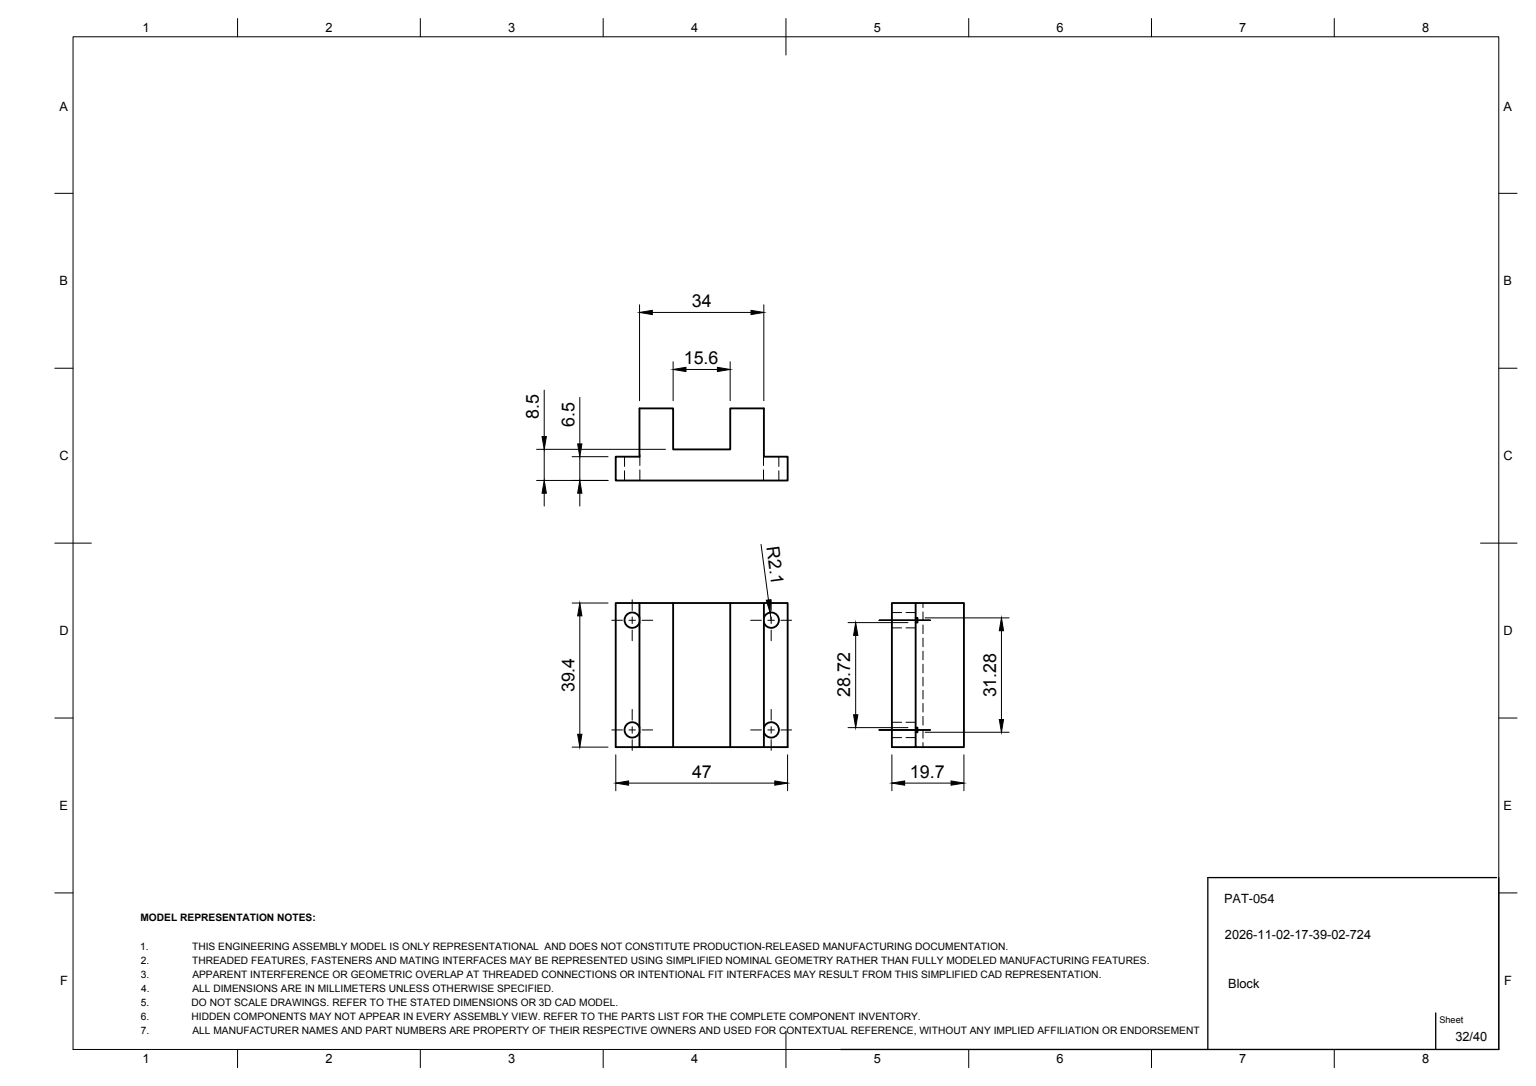
ISO-10303-21;
HEADER;
/* Generated by software containing ST-Developer
 * from STEP Tools, Inc. (www.steptools.com) 
 */

FILE_DESCRIPTION(
/* description */ ('PAT-054'),
/* implementation_level */ '2;1');

FILE_NAME(
/* name */ 'Block.step',
/* time_stamp */ '2026-10-29T16:38:13-07:00',
/* author */ (''),
/* organization */ (''),
/* preprocessor_version */ 'ST-DEVELOPER v20.2',
/* originating_system */ 'Autodesk Translation Framework v15.17.0.0',
/* authorisation */ '');

FILE_SCHEMA (('AUTOMOTIVE_DESIGN { 1 0 10303 214 3 1 1 }'));
ENDSEC;

DATA;
#10=MECHANICAL_DESIGN_GEOMETRIC_PRESENTATION_REPRESENTATION('',(#940),#33981);
#837=SHAPE_REPRESENTATION_RELATIONSHIP('SRR','None',#34214,#881);
#881=ADVANCED_BREP_SHAPE_REPRESENTATION('',(#998),#33962);
#940=STYLED_ITEM('',(#34496),#998);
#998=MANIFOLD_SOLID_BREP('Body1',#13052);
#1185=FACE_BOUND('',#2860,.T.);
#1186=FACE_BOUND('',#2861,.T.);
#1187=FACE_BOUND('',#2862,.T.);
#1188=FACE_BOUND('',#2863,.T.);
#1437=PLANE('',#14326);
#1438=PLANE('',#14332);
#1439=PLANE('',#14338);
#1440=PLANE('',#14344);
#1441=PLANE('',#14350);
#1442=PLANE('',#14351);
#1443=PLANE('',#14352);
#1444=PLANE('',#14353);
#1445=PLANE('',#14354);
#1446=PLANE('',#14355);
#1447=PLANE('',#14356);
#1448=PLANE('',#14357);
#1449=PLANE('',#14358);
#1450=PLANE('',#14359);
#1451=PLANE('',#14360);
#1452=PLANE('',#14361);
#1453=PLANE('',#14362);
#1454=PLANE('',#14363);
#1950=FACE_OUTER_BOUND('',#2846,.T.);
#1951=FACE_OUTER_BOUND('',#2847,.T.);
#1952=FACE_OUTER_BOUND('',#2848,.T.);
#1953=FACE_OUTER_BOUND('',#2849,.T.);
#1954=FACE_OUTER_BOUND('',#2850,.T.);
#1955=FACE_OUTER_BOUND('',#2851,.T.);
#1956=FACE_OUTER_BOUND('',#2852,.T.);
#1957=FACE_OUTER_BOUND('',#2853,.T.);
#1958=FACE_OUTER_BOUND('',#2854,.T.);
#1959=FACE_OUTER_BOUND('',#2855,.T.);
#1960=FACE_OUTER_BOUND('',#2856,.T.);
#1961=FACE_OUTER_BOUND('',#2857,.T.);
#1962=FACE_OUTER_BOUND('',#2858,.T.);
#1963=FACE_OUTER_BOUND('',#2859,.T.);
#1964=FACE_OUTER_BOUND('',#2864,.T.);
#1965=FACE_OUTER_BOUND('',#2865,.T.);
#1966=FACE_OUTER_BOUND('',#2866,.T.);
#1967=FACE_OUTER_BOUND('',#2867,.T.);
#1968=FACE_OUTER_BOUND('',#2868,.T.);
#1969=FACE_OUTER_BOUND('',#2869,.T.);
#1970=FACE_OUTER_BOUND('',#2870,.T.);
#1971=FACE_OUTER_BOUND('',#2871,.T.);
#2846=EDGE_LOOP('',(#10229,#10230));
#2847=EDGE_LOOP('',(#10231,#10232,#10233,#10234,#10235,#10236,#10237,#10238));
#2848=EDGE_LOOP('',(#10239,#10240));
#2849=EDGE_LOOP('',(#10241,#10242,#10243,#10244,#10245,#10246,#10247,#10248));
#2850=EDGE_LOOP('',(#10249,#10250));
#2851=EDGE_LOOP('',(#10251,#10252,#10253,#10254,#10255,#10256,#10257,#10258));
#2852=EDGE_LOOP('',(#10259,#10260));
#2853=EDGE_LOOP('',(#10261,#10262,#10263,#10264,#10265,#10266,#10267,#10268));
#2854=EDGE_LOOP('',(#10269,#10270,#10271,#10272,#10273,#10274,#10275,#10276,
#10277,#10278,#10279,#10280));
#2855=EDGE_LOOP('',(#10281,#10282,#10283,#10284,#10285,#10286,#10287,#10288,
#10289,#10290,#10291,#10292));
#2856=EDGE_LOOP('',(#10293,#10294,#10295,#10296,#10297,#10298,#10299,#10300,
#10301,#10302,#10303,#10304));
#2857=EDGE_LOOP('',(#10305,#10306,#10307,#10308,#10309,#10310,#10311,#10312,
#10313,#10314));
#2858=EDGE_LOOP('',(#10315,#10316,#10317,#10318));
#2859=EDGE_LOOP('',(#10319,#10320,#10321,#10322));
#2860=EDGE_LOOP('',(#10323));
#2861=EDGE_LOOP('',(#10324));
#2862=EDGE_LOOP('',(#10325));
#2863=EDGE_LOOP('',(#10326));
#2864=EDGE_LOOP('',(#10327,#10328,#10329,#10330));
#2865=EDGE_LOOP('',(#10331,#10332,#10333,#10334,#10335,#10336,#10337,#10338,
#10339,#10340));
#2866=EDGE_LOOP('',(#10341,#10342,#10343,#10344));
#2867=EDGE_LOOP('',(#10345,#10346,#10347,#10348));
#2868=EDGE_LOOP('',(#10349,#10350,#10351,#10352));
#2869=EDGE_LOOP('',(#10353,#10354,#10355,#10356));
#2870=EDGE_LOOP('',(#10357,#10358,#10359,#10360));
#2871=EDGE_LOOP('',(#10361,#10362,#10363,#10364,#10365,#10366,#10367,#10368,
#10369,#10370,#10371,#10372));
#3726=LINE('',#21005,#4660);
#3727=LINE('',#21009,#4661);
#3728=LINE('',#21013,#4662);
#3729=LINE('',#21017,#4663);
#3730=LINE('',#21021,#4664);
#3731=LINE('',#21025,#4665);
#3732=LINE('',#21029,#4666);
#3733=LINE('',#21033,#4667);
#3734=LINE('',#21037,#4668);
#3735=LINE('',#21041,#4669);
#3736=LINE('',#21045,#4670);
#3737=LINE('',#21049,#4671);
#3738=LINE('',#21053,#4672);
#3739=LINE('',#21057,#4673);
#3740=LINE('',#21061,#4674);
#3741=LINE('',#21065,#4675);
#3742=LINE('',#21067,#4676);
#3743=LINE('',#21069,#4677);
#3744=LINE('',#21071,#4678);
#3745=LINE('',#21073,#4679);
#3746=LINE('',#21075,#4680);
#3747=LINE('',#21076,#4681);
#3748=LINE('',#21078,#4682);
#3749=LINE('',#21080,#4683);
#3750=LINE('',#21082,#4684);
#3751=LINE('',#21084,#4685);
#3752=LINE('',#21086,#4686);
#3753=LINE('',#21087,#4687);
#3754=LINE('',#21090,#4688);
#3755=LINE('',#21092,#4689);
#3756=LINE('',#21094,#4690);
#3757=LINE('',#21096,#4691);
#3758=LINE('',#21097,#4692);
#3759=LINE('',#21099,#4693);
#3760=LINE('',#21101,#4694);
#3761=LINE('',#21103,#4695);
#3762=LINE('',#21105,#4696);
#3763=LINE('',#21106,#4697);
#3764=LINE('',#21109,#4698);
#3765=LINE('',#21110,#4699);
#3766=LINE('',#21113,#4700);
#3767=LINE('',#21114,#4701);
#3768=LINE('',#21117,#4702);
#3769=LINE('',#21118,#4703);
#3770=LINE('',#21121,#4704);
#3771=LINE('',#21122,#4705);
#3772=LINE('',#21124,#4706);
#3773=LINE('',#21127,#4707);
#3774=LINE('',#21128,#4708);
#3775=LINE('',#21131,#4709);
#3776=LINE('',#21132,#4710);
#3777=LINE('',#21135,#4711);
#3778=LINE('',#21136,#4712);
#3779=LINE('',#21139,#4713);
#3780=LINE('',#21140,#4714);
#3781=LINE('',#21142,#4715);
#4660=VECTOR('',#16915,1.);
#4661=VECTOR('',#16920,1.);
#4662=VECTOR('',#16923,0.21);
#4663=VECTOR('',#16928,1.);
#4664=VECTOR('',#16931,1.);
#4665=VECTOR('',#16936,1.);
#4666=VECTOR('',#16939,0.21);
#4667=VECTOR('',#16944,1.);
#4668=VECTOR('',#16947,1.);
#4669=VECTOR('',#16952,1.);
#4670=VECTOR('',#16955,0.21);
#4671=VECTOR('',#16960,1.);
#4672=VECTOR('',#16963,1.);
#4673=VECTOR('',#16968,1.);
#4674=VECTOR('',#16971,0.21);
#4675=VECTOR('',#16976,1.);
#4676=VECTOR('',#16979,1.);
#4677=VECTOR('',#16980,1.);
#4678=VECTOR('',#16981,1.);
#4679=VECTOR('',#16982,1.);
#4680=VECTOR('',#16983,1.);
#4681=VECTOR('',#16984,1.);
#4682=VECTOR('',#16987,1.);
#4683=VECTOR('',#16988,1.);
#4684=VECTOR('',#16989,1.);
#4685=VECTOR('',#16990,1.);
#4686=VECTOR('',#16991,1.);
#4687=VECTOR('',#16992,1.);
#4688=VECTOR('',#16995,1.);
#4689=VECTOR('',#16996,1.);
#4690=VECTOR('',#16997,1.);
#4691=VECTOR('',#16998,1.);
#4692=VECTOR('',#16999,1.);
#4693=VECTOR('',#17000,1.);
#4694=VECTOR('',#17001,1.);
#4695=VECTOR('',#17002,1.);
#4696=VECTOR('',#17003,1.);
#4697=VECTOR('',#17004,1.);
#4698=VECTOR('',#17007,1.);
#4699=VECTOR('',#17008,1.);
#4700=VECTOR('',#17011,1.);
#4701=VECTOR('',#17012,1.);
#4702=VECTOR('',#17015,1.);
#4703=VECTOR('',#17016,1.);
#4704=VECTOR('',#17019,1.);
#4705=VECTOR('',#17020,1.);
#4706=VECTOR('',#17023,1.);
#4707=VECTOR('',#17026,1.);
#4708=VECTOR('',#17027,1.);
#4709=VECTOR('',#17030,1.);
#4710=VECTOR('',#17031,1.);
#4711=VECTOR('',#17034,1.);
#4712=VECTOR('',#17035,1.);
#4713=VECTOR('',#17038,1.);
#4714=VECTOR('',#17039,1.);
#4715=VECTOR('',#17042,1.);
#5452=CIRCLE('',#14327,0.21);
#5453=CIRCLE('',#14329,0.21);
#5454=CIRCLE('',#14330,0.21);
#5455=CIRCLE('',#14331,0.21);
#5456=CIRCLE('',#14333,0.21);
#5457=CIRCLE('',#14335,0.21);
#5458=CIRCLE('',#14336,0.21);
#5459=CIRCLE('',#14337,0.21);
#5460=CIRCLE('',#14339,0.21);
#5461=CIRCLE('',#14341,0.21);
#5462=CIRCLE('',#14342,0.21);
#5463=CIRCLE('',#14343,0.21);
#5464=CIRCLE('',#14345,0.21);
#5465=CIRCLE('',#14347,0.21);
#5466=CIRCLE('',#14348,0.21);
#5467=CIRCLE('',#14349,0.21);
#6166=VERTEX_POINT('',#21003);
#6167=VERTEX_POINT('',#21004);
#6168=VERTEX_POINT('',#21008);
#6169=VERTEX_POINT('',#21010);
#6170=VERTEX_POINT('',#21012);
#6171=VERTEX_POINT('',#21015);
#6172=VERTEX_POINT('',#21019);
#6173=VERTEX_POINT('',#21020);
#6174=VERTEX_POINT('',#21024);
#6175=VERTEX_POINT('',#21026);
#6176=VERTEX_POINT('',#21028);
#6177=VERTEX_POINT('',#21031);
#6178=VERTEX_POINT('',#21035);
#6179=VERTEX_POINT('',#21036);
#6180=VERTEX_POINT('',#21040);
#6181=VERTEX_POINT('',#21042);
#6182=VERTEX_POINT('',#21044);
#6183=VERTEX_POINT('',#21047);
#6184=VERTEX_POINT('',#21051);
#6185=VERTEX_POINT('',#21052);
#6186=VERTEX_POINT('',#21056);
#6187=VERTEX_POINT('',#21058);
#6188=VERTEX_POINT('',#21060);
#6189=VERTEX_POINT('',#21063);
#6190=VERTEX_POINT('',#21068);
#6191=VERTEX_POINT('',#21070);
#6192=VERTEX_POINT('',#21072);
#6193=VERTEX_POINT('',#21074);
#6194=VERTEX_POINT('',#21079);
#6195=VERTEX_POINT('',#21081);
#6196=VERTEX_POINT('',#21083);
#6197=VERTEX_POINT('',#21085);
#6198=VERTEX_POINT('',#21089);
#6199=VERTEX_POINT('',#21091);
#6200=VERTEX_POINT('',#21093);
#6201=VERTEX_POINT('',#21095);
#6202=VERTEX_POINT('',#21098);
#6203=VERTEX_POINT('',#21100);
#6204=VERTEX_POINT('',#21102);
#6205=VERTEX_POINT('',#21104);
#6206=VERTEX_POINT('',#21108);
#6207=VERTEX_POINT('',#21112);
#6208=VERTEX_POINT('',#21116);
#6209=VERTEX_POINT('',#21120);
#6210=VERTEX_POINT('',#21126);
#6211=VERTEX_POINT('',#21130);
#6212=VERTEX_POINT('',#21134);
#6213=VERTEX_POINT('',#21138);
#7614=EDGE_CURVE('',#6166,#6167,#3726,.T.);
#7615=EDGE_CURVE('',#6166,#6167,#5452,.T.);
#7616=EDGE_CURVE('',#6168,#6166,#3727,.T.);
#7617=EDGE_CURVE('',#6169,#6168,#5453,.T.);
#7618=EDGE_CURVE('',#6169,#6170,#3728,.T.);
#7619=EDGE_CURVE('',#6170,#6170,#5454,.T.);
#7620=EDGE_CURVE('',#6171,#6169,#5455,.T.);
#7621=EDGE_CURVE('',#6167,#6171,#3729,.T.);
#7622=EDGE_CURVE('',#6172,#6173,#3730,.T.);
#7623=EDGE_CURVE('',#6172,#6173,#5456,.T.);
#7624=EDGE_CURVE('',#6174,#6172,#3731,.T.);
#7625=EDGE_CURVE('',#6175,#6174,#5457,.T.);
#7626=EDGE_CURVE('',#6175,#6176,#3732,.T.);
#7627=EDGE_CURVE('',#6176,#6176,#5458,.T.);
#7628=EDGE_CURVE('',#6177,#6175,#5459,.T.);
#7629=EDGE_CURVE('',#6173,#6177,#3733,.T.);
#7630=EDGE_CURVE('',#6178,#6179,#3734,.T.);
#7631=EDGE_CURVE('',#6178,#6179,#5460,.T.);
#7632=EDGE_CURVE('',#6180,#6178,#3735,.T.);
#7633=EDGE_CURVE('',#6181,#6180,#5461,.T.);
#7634=EDGE_CURVE('',#6181,#6182,#3736,.T.);
#7635=EDGE_CURVE('',#6182,#6182,#5462,.T.);
#7636=EDGE_CURVE('',#6183,#6181,#5463,.T.);
#7637=EDGE_CURVE('',#6179,#6183,#3737,.T.);
#7638=EDGE_CURVE('',#6184,#6185,#3738,.T.);
#7639=EDGE_CURVE('',#6184,#6185,#5464,.T.);
#7640=EDGE_CURVE('',#6186,#6184,#3739,.T.);
#7641=EDGE_CURVE('',#6187,#6186,#5465,.T.);
#7642=EDGE_CURVE('',#6187,#6188,#3740,.T.);
#7643=EDGE_CURVE('',#6188,#6188,#5466,.T.);
#7644=EDGE_CURVE('',#6189,#6187,#5467,.T.);
#7645=EDGE_CURVE('',#6185,#6189,#3741,.T.);
#7646=EDGE_CURVE('',#6171,#6180,#3742,.T.);
#7647=EDGE_CURVE('',#6183,#6190,#3743,.T.);
#7648=EDGE_CURVE('',#6191,#6190,#3744,.T.);
#7649=EDGE_CURVE('',#6191,#6192,#3745,.T.);
#7650=EDGE_CURVE('',#6193,#6192,#3746,.T.);
#7651=EDGE_CURVE('',#6193,#6168,#3747,.T.);
#7652=EDGE_CURVE('',#6177,#6186,#3748,.T.);
#7653=EDGE_CURVE('',#6189,#6194,#3749,.T.);
#7654=EDGE_CURVE('',#6195,#6194,#3750,.T.);
#7655=EDGE_CURVE('',#6196,#6195,#3751,.T.);
#7656=EDGE_CURVE('',#6197,#6196,#3752,.T.);
#7657=EDGE_CURVE('',#6197,#6174,#3753,.T.);
#7658=EDGE_CURVE('',#6190,#6198,#3754,.T.);
#7659=EDGE_CURVE('',#6198,#6199,#3755,.T.);
#7660=EDGE_CURVE('',#6199,#6200,#3756,.T.);
#7661=EDGE_CURVE('',#6200,#6201,#3757,.T.);
#7662=EDGE_CURVE('',#6201,#6197,#3758,.T.);
#7663=EDGE_CURVE('',#6196,#6202,#3759,.T.);
#7664=EDGE_CURVE('',#6202,#6203,#3760,.T.);
#7665=EDGE_CURVE('',#6203,#6204,#3761,.T.);
#7666=EDGE_CURVE('',#6204,#6205,#3762,.T.);
#7667=EDGE_CURVE('',#6205,#6191,#3763,.T.);
#7668=EDGE_CURVE('',#6206,#6193,#3764,.T.);
#7669=EDGE_CURVE('',#6198,#6206,#3765,.T.);
#7670=EDGE_CURVE('',#6207,#6206,#3766,.T.);
#7671=EDGE_CURVE('',#6199,#6207,#3767,.T.);
#7672=EDGE_CURVE('',#6208,#6207,#3768,.T.);
#7673=EDGE_CURVE('',#6200,#6208,#3769,.T.);
#7674=EDGE_CURVE('',#6209,#6208,#3770,.T.);
#7675=EDGE_CURVE('',#6201,#6209,#3771,.T.);
#7676=EDGE_CURVE('',#6194,#6209,#3772,.T.);
#7677=EDGE_CURVE('',#6210,#6195,#3773,.T.);
#7678=EDGE_CURVE('',#6202,#6210,#3774,.T.);
#7679=EDGE_CURVE('',#6211,#6210,#3775,.T.);
#7680=EDGE_CURVE('',#6203,#6211,#3776,.T.);
#7681=EDGE_CURVE('',#6212,#6211,#3777,.T.);
#7682=EDGE_CURVE('',#6204,#6212,#3778,.T.);
#7683=EDGE_CURVE('',#6213,#6212,#3779,.T.);
#7684=EDGE_CURVE('',#6205,#6213,#3780,.T.);
#7685=EDGE_CURVE('',#6192,#6213,#3781,.T.);
#10229=ORIENTED_EDGE('',*,*,#7614,.F.);
#10230=ORIENTED_EDGE('',*,*,#7615,.T.);
#10231=ORIENTED_EDGE('',*,*,#7616,.F.);
#10232=ORIENTED_EDGE('',*,*,#7617,.F.);
#10233=ORIENTED_EDGE('',*,*,#7618,.T.);
#10234=ORIENTED_EDGE('',*,*,#7619,.F.);
#10235=ORIENTED_EDGE('',*,*,#7618,.F.);
#10236=ORIENTED_EDGE('',*,*,#7620,.F.);
#10237=ORIENTED_EDGE('',*,*,#7621,.F.);
#10238=ORIENTED_EDGE('',*,*,#7615,.F.);
#10239=ORIENTED_EDGE('',*,*,#7622,.F.);
#10240=ORIENTED_EDGE('',*,*,#7623,.T.);
#10241=ORIENTED_EDGE('',*,*,#7624,.F.);
#10242=ORIENTED_EDGE('',*,*,#7625,.F.);
#10243=ORIENTED_EDGE('',*,*,#7626,.T.);
#10244=ORIENTED_EDGE('',*,*,#7627,.F.);
#10245=ORIENTED_EDGE('',*,*,#7626,.F.);
#10246=ORIENTED_EDGE('',*,*,#7628,.F.);
#10247=ORIENTED_EDGE('',*,*,#7629,.F.);
#10248=ORIENTED_EDGE('',*,*,#7623,.F.);
#10249=ORIENTED_EDGE('',*,*,#7630,.F.);
#10250=ORIENTED_EDGE('',*,*,#7631,.T.);
#10251=ORIENTED_EDGE('',*,*,#7632,.F.);
#10252=ORIENTED_EDGE('',*,*,#7633,.F.);
#10253=ORIENTED_EDGE('',*,*,#7634,.T.);
#10254=ORIENTED_EDGE('',*,*,#7635,.F.);
#10255=ORIENTED_EDGE('',*,*,#7634,.F.);
#10256=ORIENTED_EDGE('',*,*,#7636,.F.);
#10257=ORIENTED_EDGE('',*,*,#7637,.F.);
#10258=ORIENTED_EDGE('',*,*,#7631,.F.);
#10259=ORIENTED_EDGE('',*,*,#7638,.F.);
#10260=ORIENTED_EDGE('',*,*,#7639,.T.);
#10261=ORIENTED_EDGE('',*,*,#7640,.F.);
#10262=ORIENTED_EDGE('',*,*,#7641,.F.);
#10263=ORIENTED_EDGE('',*,*,#7642,.T.);
#10264=ORIENTED_EDGE('',*,*,#7643,.F.);
#10265=ORIENTED_EDGE('',*,*,#7642,.F.);
#10266=ORIENTED_EDGE('',*,*,#7644,.F.);
#10267=ORIENTED_EDGE('',*,*,#7645,.F.);
#10268=ORIENTED_EDGE('',*,*,#7639,.F.);
#10269=ORIENTED_EDGE('',*,*,#7616,.T.);
#10270=ORIENTED_EDGE('',*,*,#7614,.T.);
#10271=ORIENTED_EDGE('',*,*,#7621,.T.);
#10272=ORIENTED_EDGE('',*,*,#7646,.T.);
#10273=ORIENTED_EDGE('',*,*,#7632,.T.);
#10274=ORIENTED_EDGE('',*,*,#7630,.T.);
#10275=ORIENTED_EDGE('',*,*,#7637,.T.);
#10276=ORIENTED_EDGE('',*,*,#7647,.T.);
#10277=ORIENTED_EDGE('',*,*,#7648,.F.);
#10278=ORIENTED_EDGE('',*,*,#7649,.T.);
#10279=ORIENTED_EDGE('',*,*,#7650,.F.);
#10280=ORIENTED_EDGE('',*,*,#7651,.T.);
#10281=ORIENTED_EDGE('',*,*,#7624,.T.);
#10282=ORIENTED_EDGE('',*,*,#7622,.T.);
#10283=ORIENTED_EDGE('',*,*,#7629,.T.);
#10284=ORIENTED_EDGE('',*,*,#7652,.T.);
#10285=ORIENTED_EDGE('',*,*,#7640,.T.);
#10286=ORIENTED_EDGE('',*,*,#7638,.T.);
#10287=ORIENTED_EDGE('',*,*,#7645,.T.);
#10288=ORIENTED_EDGE('',*,*,#7653,.T.);
#10289=ORIENTED_EDGE('',*,*,#7654,.F.);
#10290=ORIENTED_EDGE('',*,*,#7655,.F.);
#10291=ORIENTED_EDGE('',*,*,#7656,.F.);
#10292=ORIENTED_EDGE('',*,*,#7657,.T.);
#10293=ORIENTED_EDGE('',*,*,#7648,.T.);
#10294=ORIENTED_EDGE('',*,*,#7658,.T.);
#10295=ORIENTED_EDGE('',*,*,#7659,.T.);
#10296=ORIENTED_EDGE('',*,*,#7660,.T.);
#10297=ORIENTED_EDGE('',*,*,#7661,.T.);
#10298=ORIENTED_EDGE('',*,*,#7662,.T.);
#10299=ORIENTED_EDGE('',*,*,#7656,.T.);
#10300=ORIENTED_EDGE('',*,*,#7663,.T.);
#10301=ORIENTED_EDGE('',*,*,#7664,.T.);
#10302=ORIENTED_EDGE('',*,*,#7665,.T.);
#10303=ORIENTED_EDGE('',*,*,#7666,.T.);
#10304=ORIENTED_EDGE('',*,*,#7667,.T.);
#10305=ORIENTED_EDGE('',*,*,#7620,.T.);
#10306=ORIENTED_EDGE('',*,*,#7617,.T.);
#10307=ORIENTED_EDGE('',*,*,#7651,.F.);
#10308=ORIENTED_EDGE('',*,*,#7668,.F.);
#10309=ORIENTED_EDGE('',*,*,#7669,.F.);
#10310=ORIENTED_EDGE('',*,*,#7658,.F.);
#10311=ORIENTED_EDGE('',*,*,#7647,.F.);
#10312=ORIENTED_EDGE('',*,*,#7636,.T.);
#10313=ORIENTED_EDGE('',*,*,#7633,.T.);
#10314=ORIENTED_EDGE('',*,*,#7646,.F.);
#10315=ORIENTED_EDGE('',*,*,#7669,.T.);
#10316=ORIENTED_EDGE('',*,*,#7670,.F.);
#10317=ORIENTED_EDGE('',*,*,#7671,.F.);
#10318=ORIENTED_EDGE('',*,*,#7659,.F.);
#10319=ORIENTED_EDGE('',*,*,#7671,.T.);
#10320=ORIENTED_EDGE('',*,*,#7672,.F.);
#10321=ORIENTED_EDGE('',*,*,#7673,.F.);
#10322=ORIENTED_EDGE('',*,*,#7660,.F.);
#10323=ORIENTED_EDGE('',*,*,#7619,.T.);
#10324=ORIENTED_EDGE('',*,*,#7627,.T.);
#10325=ORIENTED_EDGE('',*,*,#7635,.T.);
#10326=ORIENTED_EDGE('',*,*,#7643,.T.);
#10327=ORIENTED_EDGE('',*,*,#7673,.T.);
#10328=ORIENTED_EDGE('',*,*,#7674,.F.);
#10329=ORIENTED_EDGE('',*,*,#7675,.F.);
#10330=ORIENTED_EDGE('',*,*,#7661,.F.);
#10331=ORIENTED_EDGE('',*,*,#7628,.T.);
#10332=ORIENTED_EDGE('',*,*,#7625,.T.);
#10333=ORIENTED_EDGE('',*,*,#7657,.F.);
#10334=ORIENTED_EDGE('',*,*,#7662,.F.);
#10335=ORIENTED_EDGE('',*,*,#7675,.T.);
#10336=ORIENTED_EDGE('',*,*,#7676,.F.);
#10337=ORIENTED_EDGE('',*,*,#7653,.F.);
#10338=ORIENTED_EDGE('',*,*,#7644,.T.);
#10339=ORIENTED_EDGE('',*,*,#7641,.T.);
#10340=ORIENTED_EDGE('',*,*,#7652,.F.);
#10341=ORIENTED_EDGE('',*,*,#7655,.T.);
#10342=ORIENTED_EDGE('',*,*,#7677,.F.);
#10343=ORIENTED_EDGE('',*,*,#7678,.F.);
#10344=ORIENTED_EDGE('',*,*,#7663,.F.);
#10345=ORIENTED_EDGE('',*,*,#7678,.T.);
#10346=ORIENTED_EDGE('',*,*,#7679,.F.);
#10347=ORIENTED_EDGE('',*,*,#7680,.F.);
#10348=ORIENTED_EDGE('',*,*,#7664,.F.);
#10349=ORIENTED_EDGE('',*,*,#7680,.T.);
#10350=ORIENTED_EDGE('',*,*,#7681,.F.);
#10351=ORIENTED_EDGE('',*,*,#7682,.F.);
#10352=ORIENTED_EDGE('',*,*,#7665,.F.);
#10353=ORIENTED_EDGE('',*,*,#7682,.T.);
#10354=ORIENTED_EDGE('',*,*,#7683,.F.);
#10355=ORIENTED_EDGE('',*,*,#7684,.F.);
#10356=ORIENTED_EDGE('',*,*,#7666,.F.);
#10357=ORIENTED_EDGE('',*,*,#7684,.T.);
#10358=ORIENTED_EDGE('',*,*,#7685,.F.);
#10359=ORIENTED_EDGE('',*,*,#7649,.F.);
#10360=ORIENTED_EDGE('',*,*,#7667,.F.);
#10361=ORIENTED_EDGE('',*,*,#7650,.T.);
#10362=ORIENTED_EDGE('',*,*,#7685,.T.);
#10363=ORIENTED_EDGE('',*,*,#7683,.T.);
#10364=ORIENTED_EDGE('',*,*,#7681,.T.);
#10365=ORIENTED_EDGE('',*,*,#7679,.T.);
#10366=ORIENTED_EDGE('',*,*,#7677,.T.);
#10367=ORIENTED_EDGE('',*,*,#7654,.T.);
#10368=ORIENTED_EDGE('',*,*,#7676,.T.);
#10369=ORIENTED_EDGE('',*,*,#7674,.T.);
#10370=ORIENTED_EDGE('',*,*,#7672,.T.);
#10371=ORIENTED_EDGE('',*,*,#7670,.T.);
#10372=ORIENTED_EDGE('',*,*,#7668,.T.);
#12099=CYLINDRICAL_SURFACE('',#14328,0.21);
#12100=CYLINDRICAL_SURFACE('',#14334,0.21);
#12101=CYLINDRICAL_SURFACE('',#14340,0.21);
#12102=CYLINDRICAL_SURFACE('',#14346,0.21);
#12662=ADVANCED_FACE('',(#1950),#1437,.T.);
#12663=ADVANCED_FACE('',(#1951),#12099,.F.);
#12664=ADVANCED_FACE('',(#1952),#1438,.T.);
#12665=ADVANCED_FACE('',(#1953),#12100,.F.);
#12666=ADVANCED_FACE('',(#1954),#1439,.T.);
#12667=ADVANCED_FACE('',(#1955),#12101,.F.);
#12668=ADVANCED_FACE('',(#1956),#1440,.T.);
#12669=ADVANCED_FACE('',(#1957),#12102,.F.);
#12670=ADVANCED_FACE('',(#1958),#1441,.T.);
#12671=ADVANCED_FACE('',(#1959),#1442,.T.);
#12672=ADVANCED_FACE('',(#1960),#1443,.T.);
#12673=ADVANCED_FACE('',(#1961),#1444,.T.);
#12674=ADVANCED_FACE('',(#1962),#1445,.T.);
#12675=ADVANCED_FACE('',(#1963,#1185,#1186,#1187,#1188),#1446,.T.);
#12676=ADVANCED_FACE('',(#1964),#1447,.T.);
#12677=ADVANCED_FACE('',(#1965),#1448,.T.);
#12678=ADVANCED_FACE('',(#1966),#1449,.T.);
#12679=ADVANCED_FACE('',(#1967),#1450,.T.);
#12680=ADVANCED_FACE('',(#1968),#1451,.T.);
#12681=ADVANCED_FACE('',(#1969),#1452,.T.);
#12682=ADVANCED_FACE('',(#1970),#1453,.T.);
#12683=ADVANCED_FACE('',(#1971),#1454,.T.);
#13052=CLOSED_SHELL('',(#12662,#12663,#12664,#12665,#12666,#12667,#12668,
#12669,#12670,#12671,#12672,#12673,#12674,#12675,#12676,#12677,#12678,#12679,
#12680,#12681,#12682,#12683));
#14325=AXIS2_PLACEMENT_3D('',#21001,#16911,#16912);
#14326=AXIS2_PLACEMENT_3D('',#21002,#16913,#16914);
#14327=AXIS2_PLACEMENT_3D('',#21006,#16916,#16917);
#14328=AXIS2_PLACEMENT_3D('',#21007,#16918,#16919);
#14329=AXIS2_PLACEMENT_3D('',#21011,#16921,#16922);
#14330=AXIS2_PLACEMENT_3D('',#21014,#16924,#16925);
#14331=AXIS2_PLACEMENT_3D('',#21016,#16926,#16927);
#14332=AXIS2_PLACEMENT_3D('',#21018,#16929,#16930);
#14333=AXIS2_PLACEMENT_3D('',#21022,#16932,#16933);
#14334=AXIS2_PLACEMENT_3D('',#21023,#16934,#16935);
#14335=AXIS2_PLACEMENT_3D('',#21027,#16937,#16938);
#14336=AXIS2_PLACEMENT_3D('',#21030,#16940,#16941);
#14337=AXIS2_PLACEMENT_3D('',#21032,#16942,#16943);
#14338=AXIS2_PLACEMENT_3D('',#21034,#16945,#16946);
#14339=AXIS2_PLACEMENT_3D('',#21038,#16948,#16949);
#14340=AXIS2_PLACEMENT_3D('',#21039,#16950,#16951);
#14341=AXIS2_PLACEMENT_3D('',#21043,#16953,#16954);
#14342=AXIS2_PLACEMENT_3D('',#21046,#16956,#16957);
#14343=AXIS2_PLACEMENT_3D('',#21048,#16958,#16959);
#14344=AXIS2_PLACEMENT_3D('',#21050,#16961,#16962);
#14345=AXIS2_PLACEMENT_3D('',#21054,#16964,#16965);
#14346=AXIS2_PLACEMENT_3D('',#21055,#16966,#16967);
#14347=AXIS2_PLACEMENT_3D('',#21059,#16969,#16970);
#14348=AXIS2_PLACEMENT_3D('',#21062,#16972,#16973);
#14349=AXIS2_PLACEMENT_3D('',#21064,#16974,#16975);
#14350=AXIS2_PLACEMENT_3D('',#21066,#16977,#16978);
#14351=AXIS2_PLACEMENT_3D('',#21077,#16985,#16986);
#14352=AXIS2_PLACEMENT_3D('',#21088,#16993,#16994);
#14353=AXIS2_PLACEMENT_3D('',#21107,#17005,#17006);
#14354=AXIS2_PLACEMENT_3D('',#21111,#17009,#17010);
#14355=AXIS2_PLACEMENT_3D('',#21115,#17013,#17014);
#14356=AXIS2_PLACEMENT_3D('',#21119,#17017,#17018);
#14357=AXIS2_PLACEMENT_3D('',#21123,#17021,#17022);
#14358=AXIS2_PLACEMENT_3D('',#21125,#17024,#17025);
#14359=AXIS2_PLACEMENT_3D('',#21129,#17028,#17029);
#14360=AXIS2_PLACEMENT_3D('',#21133,#17032,#17033);
#14361=AXIS2_PLACEMENT_3D('',#21137,#17036,#17037);
#14362=AXIS2_PLACEMENT_3D('',#21141,#17040,#17041);
#14363=AXIS2_PLACEMENT_3D('',#21143,#17043,#17044);
#16911=DIRECTION('axis',(0.,0.,1.));
#16912=DIRECTION('refdir',(1.,0.,0.));
#16913=DIRECTION('center_axis',(0.,0.,1.));
#16914=DIRECTION('ref_axis',(1.,0.,0.));
#16915=DIRECTION('',(-1.,0.,0.));
#16916=DIRECTION('center_axis',(0.,0.,1.));
#16917=DIRECTION('ref_axis',(1.,0.,0.));
#16918=DIRECTION('center_axis',(0.,0.,1.));
#16919=DIRECTION('ref_axis',(1.,0.,0.));
#16920=DIRECTION('',(0.,0.,-1.));
#16921=DIRECTION('center_axis',(0.,0.,1.));
#16922=DIRECTION('ref_axis',(1.,0.,0.));
#16923=DIRECTION('',(0.,0.,1.));
#16924=DIRECTION('center_axis',(0.,0.,-1.));
#16925=DIRECTION('ref_axis',(1.,0.,0.));
#16926=DIRECTION('center_axis',(0.,0.,1.));
#16927=DIRECTION('ref_axis',(1.,0.,0.));
#16928=DIRECTION('',(0.,0.,1.));
#16929=DIRECTION('center_axis',(0.,0.,1.));
#16930=DIRECTION('ref_axis',(1.,0.,0.));
#16931=DIRECTION('',(1.,0.,0.));
#16932=DIRECTION('center_axis',(0.,0.,1.));
#16933=DIRECTION('ref_axis',(1.,0.,0.));
#16934=DIRECTION('center_axis',(0.,0.,1.));
#16935=DIRECTION('ref_axis',(1.,0.,0.));
#16936=DIRECTION('',(0.,0.,-1.));
#16937=DIRECTION('center_axis',(0.,0.,1.));
#16938=DIRECTION('ref_axis',(1.,0.,0.));
#16939=DIRECTION('',(0.,0.,1.));
#16940=DIRECTION('center_axis',(0.,0.,-1.));
#16941=DIRECTION('ref_axis',(1.,0.,0.));
#16942=DIRECTION('center_axis',(0.,0.,1.));
#16943=DIRECTION('ref_axis',(1.,0.,0.));
#16944=DIRECTION('',(0.,0.,1.));
#16945=DIRECTION('center_axis',(0.,0.,1.));
#16946=DIRECTION('ref_axis',(1.,0.,0.));
#16947=DIRECTION('',(-1.,0.,0.));
#16948=DIRECTION('center_axis',(0.,0.,1.));
#16949=DIRECTION('ref_axis',(1.,0.,0.));
#16950=DIRECTION('center_axis',(0.,0.,1.));
#16951=DIRECTION('ref_axis',(1.,0.,0.));
#16952=DIRECTION('',(0.,0.,-1.));
#16953=DIRECTION('center_axis',(0.,0.,1.));
#16954=DIRECTION('ref_axis',(1.,0.,0.));
#16955=DIRECTION('',(0.,0.,1.));
#16956=DIRECTION('center_axis',(0.,0.,-1.));
#16957=DIRECTION('ref_axis',(1.,0.,0.));
#16958=DIRECTION('center_axis',(0.,0.,1.));
#16959=DIRECTION('ref_axis',(1.,0.,0.));
#16960=DIRECTION('',(0.,0.,1.));
#16961=DIRECTION('center_axis',(0.,0.,1.));
#16962=DIRECTION('ref_axis',(1.,0.,0.));
#16963=DIRECTION('',(1.,0.,0.));
#16964=DIRECTION('center_axis',(0.,0.,1.));
#16965=DIRECTION('ref_axis',(1.,0.,0.));
#16966=DIRECTION('center_axis',(0.,0.,1.));
#16967=DIRECTION('ref_axis',(1.,0.,0.));
#16968=DIRECTION('',(0.,0.,-1.));
#16969=DIRECTION('center_axis',(0.,0.,1.));
#16970=DIRECTION('ref_axis',(1.,0.,0.));
#16971=DIRECTION('',(0.,0.,1.));
#16972=DIRECTION('center_axis',(0.,0.,-1.));
#16973=DIRECTION('ref_axis',(1.,0.,0.));
#16974=DIRECTION('center_axis',(0.,0.,1.));
#16975=DIRECTION('ref_axis',(1.,0.,0.));
#16976=DIRECTION('',(0.,0.,1.));
#16977=DIRECTION('center_axis',(0.,-1.,0.));
#16978=DIRECTION('ref_axis',(0.,0.,-1.));
#16979=DIRECTION('',(-1.,0.,0.));
#16980=DIRECTION('',(-1.,0.,0.));
#16981=DIRECTION('',(0.,0.,1.));
#16982=DIRECTION('',(1.,0.,0.));
#16983=DIRECTION('',(0.,0.,-1.));
#16984=DIRECTION('',(-1.,0.,0.));
#16985=DIRECTION('center_axis',(0.,1.,0.));
#16986=DIRECTION('ref_axis',(0.,0.,1.));
#16987=DIRECTION('',(1.,0.,0.));
#16988=DIRECTION('',(1.,0.,0.));
#16989=DIRECTION('',(0.,0.,1.));
#16990=DIRECTION('',(1.,0.,0.));
#16991=DIRECTION('',(0.,0.,-1.));
#16992=DIRECTION('',(1.,0.,0.));
#16993=DIRECTION('center_axis',(-1.,0.,0.));
#16994=DIRECTION('ref_axis',(0.,0.,1.));
#16995=DIRECTION('',(0.,-1.,0.));
#16996=DIRECTION('',(0.,0.,1.));
#16997=DIRECTION('',(0.,1.,0.));
#16998=DIRECTION('',(0.,0.,-1.));
#16999=DIRECTION('',(0.,-1.,0.));
#17000=DIRECTION('',(0.,-1.,0.));
#17001=DIRECTION('',(0.,0.,1.));
#17002=DIRECTION('',(0.,-1.,0.));
#17003=DIRECTION('',(0.,0.,-1.));
#17004=DIRECTION('',(0.,-1.,0.));
#17005=DIRECTION('center_axis',(0.,0.,-1.));
#17006=DIRECTION('ref_axis',(0.,1.,0.));
#17007=DIRECTION('',(0.,1.,0.));
#17008=DIRECTION('',(1.,0.,0.));
#17009=DIRECTION('center_axis',(0.,-1.,0.));
#17010=DIRECTION('ref_axis',(0.,0.,-1.));
#17011=DIRECTION('',(0.,0.,-1.));
#17012=DIRECTION('',(1.,0.,0.));
#17013=DIRECTION('center_axis',(0.,0.,1.));
#17014=DIRECTION('ref_axis',(0.,-1.,0.));
#17015=DIRECTION('',(0.,-1.,0.));
#17016=DIRECTION('',(1.,0.,0.));
#17017=DIRECTION('center_axis',(0.,1.,0.));
#17018=DIRECTION('ref_axis',(0.,0.,1.));
#17019=DIRECTION('',(0.,0.,1.));
#17020=DIRECTION('',(1.,0.,0.));
#17021=DIRECTION('center_axis',(0.,0.,-1.));
#17022=DIRECTION('ref_axis',(0.,1.,0.));
#17023=DIRECTION('',(0.,1.,0.));
#17024=DIRECTION('center_axis',(0.,0.,-1.));
#17025=DIRECTION('ref_axis',(0.,1.,0.));
#17026=DIRECTION('',(0.,1.,0.));
#17027=DIRECTION('',(1.,0.,0.));
#17028=DIRECTION('center_axis',(0.,-1.,0.));
#17029=DIRECTION('ref_axis',(0.,0.,-1.));
#17030=DIRECTION('',(0.,0.,-1.));
#17031=DIRECTION('',(1.,0.,0.));
#17032=DIRECTION('center_axis',(0.,0.,-1.));
#17033=DIRECTION('ref_axis',(0.,1.,0.));
#17034=DIRECTION('',(0.,1.,0.));
#17035=DIRECTION('',(1.,0.,0.));
#17036=DIRECTION('center_axis',(0.,1.,0.));
#17037=DIRECTION('ref_axis',(0.,0.,1.));
#17038=DIRECTION('',(0.,0.,1.));
#17039=DIRECTION('',(1.,0.,0.));
#17040=DIRECTION('center_axis',(0.,0.,-1.));
#17041=DIRECTION('ref_axis',(0.,1.,0.));
#17042=DIRECTION('',(0.,1.,0.));
#17043=DIRECTION('center_axis',(1.,0.,0.));
#17044=DIRECTION('ref_axis',(0.,0.,-1.));
#21001=CARTESIAN_POINT('',(0.,0.,0.));
#21002=CARTESIAN_POINT('Origin',(1.5,-1.9,1.7));
#21003=CARTESIAN_POINT('',(1.56403124237433,-1.7,1.7));
#21004=CARTESIAN_POINT('',(1.43596875762567,-1.7,1.7));
#21005=CARTESIAN_POINT('',(0.75,-1.7,1.7));
#21006=CARTESIAN_POINT('Origin',(1.5,-1.9,1.7));
#21007=CARTESIAN_POINT('Origin',(1.5,-1.9,1.7));
#21008=CARTESIAN_POINT('',(1.56403124237433,-1.7,1.75));
#21009=CARTESIAN_POINT('',(1.56403124237433,-1.7,1.7));
#21010=CARTESIAN_POINT('',(1.29,-1.9,1.75));
#21011=CARTESIAN_POINT('Origin',(1.5,-1.9,1.75));
#21012=CARTESIAN_POINT('',(1.29,-1.9,2.4));
#21013=CARTESIAN_POINT('',(1.29,-1.9,1.7));
#21014=CARTESIAN_POINT('Origin',(1.5,-1.9,2.4));
#21015=CARTESIAN_POINT('',(1.43596875762567,-1.7,1.75));
#21016=CARTESIAN_POINT('Origin',(1.5,-1.9,1.75));
#21017=CARTESIAN_POINT('',(1.43596875762567,-1.7,1.7));
#21018=CARTESIAN_POINT('Origin',(-1.5,1.9,1.7));
#21019=CARTESIAN_POINT('',(-1.56403124237433,1.7,1.7));
#21020=CARTESIAN_POINT('',(-1.43596875762567,1.7,1.7));
#21021=CARTESIAN_POINT('',(-0.75,1.7,1.7));
#21022=CARTESIAN_POINT('Origin',(-1.5,1.9,1.7));
#21023=CARTESIAN_POINT('Origin',(-1.5,1.9,1.7));
#21024=CARTESIAN_POINT('',(-1.56403124237433,1.7,1.75));
#21025=CARTESIAN_POINT('',(-1.56403124237433,1.7,1.7));
#21026=CARTESIAN_POINT('',(-1.71,1.9,1.75));
#21027=CARTESIAN_POINT('Origin',(-1.5,1.9,1.75));
#21028=CARTESIAN_POINT('',(-1.71,1.9,2.4));
#21029=CARTESIAN_POINT('',(-1.71,1.9,1.7));
#21030=CARTESIAN_POINT('Origin',(-1.5,1.9,2.4));
#21031=CARTESIAN_POINT('',(-1.43596875762567,1.7,1.75));
#21032=CARTESIAN_POINT('Origin',(-1.5,1.9,1.75));
#21033=CARTESIAN_POINT('',(-1.43596875762567,1.7,1.7));
#21034=CARTESIAN_POINT('Origin',(-1.5,-1.9,1.7));
#21035=CARTESIAN_POINT('',(-1.43596875762567,-1.7,1.7));
#21036=CARTESIAN_POINT('',(-1.56403124237433,-1.7,1.7));
#21037=CARTESIAN_POINT('',(-0.75,-1.7,1.7));
#21038=CARTESIAN_POINT('Origin',(-1.5,-1.9,1.7));
#21039=CARTESIAN_POINT('Origin',(-1.5,-1.9,1.7));
#21040=CARTESIAN_POINT('',(-1.43596875762567,-1.7,1.75));
#21041=CARTESIAN_POINT('',(-1.43596875762567,-1.7,1.7));
#21042=CARTESIAN_POINT('',(-1.71,-1.9,1.75));
#21043=CARTESIAN_POINT('Origin',(-1.5,-1.9,1.75));
#21044=CARTESIAN_POINT('',(-1.71,-1.9,2.4));
#21045=CARTESIAN_POINT('',(-1.71,-1.9,1.7));
#21046=CARTESIAN_POINT('Origin',(-1.5,-1.9,2.4));
#21047=CARTESIAN_POINT('',(-1.56403124237433,-1.7,1.75));
#21048=CARTESIAN_POINT('Origin',(-1.5,-1.9,1.75));
#21049=CARTESIAN_POINT('',(-1.56403124237433,-1.7,1.7));
#21050=CARTESIAN_POINT('Origin',(1.5,1.9,1.7));
#21051=CARTESIAN_POINT('',(1.43596875762567,1.7,1.7));
#21052=CARTESIAN_POINT('',(1.56403124237433,1.7,1.7));
#21053=CARTESIAN_POINT('',(0.75,1.7,1.7));
#21054=CARTESIAN_POINT('Origin',(1.5,1.9,1.7));
#21055=CARTESIAN_POINT('Origin',(1.5,1.9,1.7));
#21056=CARTESIAN_POINT('',(1.43596875762567,1.7,1.75));
#21057=CARTESIAN_POINT('',(1.43596875762567,1.7,1.7));
#21058=CARTESIAN_POINT('',(1.29,1.9,1.75));
#21059=CARTESIAN_POINT('Origin',(1.5,1.9,1.75));
#21060=CARTESIAN_POINT('',(1.29,1.9,2.4));
#21061=CARTESIAN_POINT('',(1.29,1.9,1.7));
#21062=CARTESIAN_POINT('Origin',(1.5,1.9,2.4));
#21063=CARTESIAN_POINT('',(1.56403124237433,1.7,1.75));
#21064=CARTESIAN_POINT('Origin',(1.5,1.9,1.75));
#21065=CARTESIAN_POINT('',(1.56403124237433,1.7,1.7));
#21066=CARTESIAN_POINT('Origin',(0.,-1.7,1.75));
#21067=CARTESIAN_POINT('',(0.,-1.7,1.75));
#21068=CARTESIAN_POINT('',(-1.97,-1.7,1.75));
#21069=CARTESIAN_POINT('',(0.,-1.7,1.75));
#21070=CARTESIAN_POINT('',(-1.97,-1.7,0.43));
#21071=CARTESIAN_POINT('',(-1.97,-1.7,1.75));
#21072=CARTESIAN_POINT('',(1.97,-1.7,0.43));
#21073=CARTESIAN_POINT('',(0.,-1.7,0.43));
#21074=CARTESIAN_POINT('',(1.97,-1.7,1.75));
#21075=CARTESIAN_POINT('',(1.97,-1.7,1.75));
#21076=CARTESIAN_POINT('',(0.,-1.7,1.75));
#21077=CARTESIAN_POINT('Origin',(0.,1.7,0.43));
#21078=CARTESIAN_POINT('',(0.,1.7,1.75));
#21079=CARTESIAN_POINT('',(1.97,1.7,1.75));
#21080=CARTESIAN_POINT('',(0.,1.7,1.75));
#21081=CARTESIAN_POINT('',(1.97,1.7,0.43));
#21082=CARTESIAN_POINT('',(1.97,1.7,0.43));
#21083=CARTESIAN_POINT('',(-1.97,1.7,0.43));
#21084=CARTESIAN_POINT('',(0.,1.7,0.43));
#21085=CARTESIAN_POINT('',(-1.97,1.7,1.75));
#21086=CARTESIAN_POINT('',(-1.97,1.7,0.43));
#21087=CARTESIAN_POINT('',(0.,1.7,1.75));
#21088=CARTESIAN_POINT('Origin',(-1.97,0.,1.415));
#21089=CARTESIAN_POINT('',(-1.97,-2.35,1.75));
#21090=CARTESIAN_POINT('',(-1.97,-2.35,1.75));
#21091=CARTESIAN_POINT('',(-1.97,-2.35,2.4));
#21092=CARTESIAN_POINT('',(-1.97,-2.35,2.4));
#21093=CARTESIAN_POINT('',(-1.97,2.35,2.4));
#21094=CARTESIAN_POINT('',(-1.97,2.35,2.4));
#21095=CARTESIAN_POINT('',(-1.97,2.35,1.75));
#21096=CARTESIAN_POINT('',(-1.97,2.35,1.75));
#21097=CARTESIAN_POINT('',(-1.97,1.7,1.75));
#21098=CARTESIAN_POINT('',(-1.97,0.78,0.43));
#21099=CARTESIAN_POINT('',(-1.97,0.78,0.43));
#21100=CARTESIAN_POINT('',(-1.97,0.78,1.55));
#21101=CARTESIAN_POINT('',(-1.97,0.78,1.55));
#21102=CARTESIAN_POINT('',(-1.97,-0.78,1.55));
#21103=CARTESIAN_POINT('',(-1.97,-0.78,1.55));
#21104=CARTESIAN_POINT('',(-1.97,-0.78,0.43));
#21105=CARTESIAN_POINT('',(-1.97,-0.78,0.43));
#21106=CARTESIAN_POINT('',(-1.97,-1.7,0.43));
#21107=CARTESIAN_POINT('Origin',(0.,-2.35,1.75));
#21108=CARTESIAN_POINT('',(1.97,-2.35,1.75));
#21109=CARTESIAN_POINT('',(1.97,-2.35,1.75));
#21110=CARTESIAN_POINT('',(0.,-2.35,1.75));
#21111=CARTESIAN_POINT('Origin',(0.,-2.35,2.4));
#21112=CARTESIAN_POINT('',(1.97,-2.35,2.4));
#21113=CARTESIAN_POINT('',(1.97,-2.35,2.4));
#21114=CARTESIAN_POINT('',(0.,-2.35,2.4));
#21115=CARTESIAN_POINT('Origin',(0.,2.35,2.4));
#21116=CARTESIAN_POINT('',(1.97,2.35,2.4));
#21117=CARTESIAN_POINT('',(1.97,2.35,2.4));
#21118=CARTESIAN_POINT('',(0.,2.35,2.4));
#21119=CARTESIAN_POINT('Origin',(0.,2.35,1.75));
#21120=CARTESIAN_POINT('',(1.97,2.35,1.75));
#21121=CARTESIAN_POINT('',(1.97,2.35,1.75));
#21122=CARTESIAN_POINT('',(0.,2.35,1.75));
#21123=CARTESIAN_POINT('Origin',(0.,1.7,1.75));
#21124=CARTESIAN_POINT('',(1.97,1.7,1.75));
#21125=CARTESIAN_POINT('Origin',(0.,0.78,0.43));
#21126=CARTESIAN_POINT('',(1.97,0.78,0.43));
#21127=CARTESIAN_POINT('',(1.97,0.78,0.43));
#21128=CARTESIAN_POINT('',(0.,0.78,0.43));
#21129=CARTESIAN_POINT('Origin',(0.,0.78,1.55));
#21130=CARTESIAN_POINT('',(1.97,0.78,1.55));
#21131=CARTESIAN_POINT('',(1.97,0.78,1.55));
#21132=CARTESIAN_POINT('',(0.,0.78,1.55));
#21133=CARTESIAN_POINT('Origin',(0.,-0.78,1.55));
#21134=CARTESIAN_POINT('',(1.97,-0.78,1.55));
#21135=CARTESIAN_POINT('',(1.97,-0.78,1.55));
#21136=CARTESIAN_POINT('',(0.,-0.78,1.55));
#21137=CARTESIAN_POINT('Origin',(0.,-0.78,0.43));
#21138=CARTESIAN_POINT('',(1.97,-0.78,0.43));
#21139=CARTESIAN_POINT('',(1.97,-0.78,0.43));
#21140=CARTESIAN_POINT('',(0.,-0.78,0.43));
#21141=CARTESIAN_POINT('Origin',(0.,-1.7,0.43));
#21142=CARTESIAN_POINT('',(1.97,-1.7,0.43));
#21143=CARTESIAN_POINT('Origin',(1.97,0.,1.415));
#33910=UNCERTAINTY_MEASURE_WITH_UNIT(LENGTH_MEASURE(0.001),#33982,
'DISTANCE_ACCURACY_VALUE',
'Maximum model space distance between geometric entities at asserted c
onnectivities');
#33929=UNCERTAINTY_MEASURE_WITH_UNIT(LENGTH_MEASURE(0.001),#33982,
'DISTANCE_ACCURACY_VALUE',
'Maximum model space distance between geometric entities at asserted c
onnectivities');
#33962=(
GEOMETRIC_REPRESENTATION_CONTEXT(3)
GLOBAL_UNCERTAINTY_ASSIGNED_CONTEXT((#33910))
GLOBAL_UNIT_ASSIGNED_CONTEXT((#33982,#33984,#33985))
REPRESENTATION_CONTEXT('','3D')
);
#33981=(
GEOMETRIC_REPRESENTATION_CONTEXT(3)
GLOBAL_UNCERTAINTY_ASSIGNED_CONTEXT((#33929))
GLOBAL_UNIT_ASSIGNED_CONTEXT((#33982,#33984,#33985))
REPRESENTATION_CONTEXT('','3D')
);
#33982=(
LENGTH_UNIT()
NAMED_UNIT(*)
SI_UNIT(.CENTI.,.METRE.)
);
#33984=(
NAMED_UNIT(*)
PLANE_ANGLE_UNIT()
SI_UNIT($,.RADIAN.)
);
#33985=(
NAMED_UNIT(*)
SI_UNIT($,.STERADIAN.)
SOLID_ANGLE_UNIT()
);
#34018=SHAPE_DEFINITION_REPRESENTATION(#34079,#34214);
#34079=PRODUCT_DEFINITION_SHAPE('',$,#34266);
#34214=SHAPE_REPRESENTATION('',(#14325),#33962);
#34233=PRODUCT_DEFINITION_CONTEXT('part definition',#34388,'design');
#34266=PRODUCT_DEFINITION('Block','Block',#34317,#34233);
#34317=PRODUCT_DEFINITION_FORMATION('',$,#34422);
#34388=APPLICATION_CONTEXT(
'Core Data for Automotive Mechanical Design Process');
#34389=PRODUCT_CONTEXT('part definition',#34388,'mechanical');
#34422=PRODUCT('Block','Block','Block',(#34389));
#34490=COLOUR_RGB('Dark Blue',0.08,0.2,0.34);
#34491=FILL_AREA_STYLE_COLOUR('',#34490);
#34492=FILL_AREA_STYLE('',(#34491));
#34493=SURFACE_STYLE_FILL_AREA(#34492);
#34494=SURFACE_SIDE_STYLE('',(#34493));
#34495=SURFACE_STYLE_USAGE(.BOTH.,#34494);
#34496=PRESENTATION_STYLE_ASSIGNMENT((#34495));
ENDSEC;
END-ISO-10303-21;
